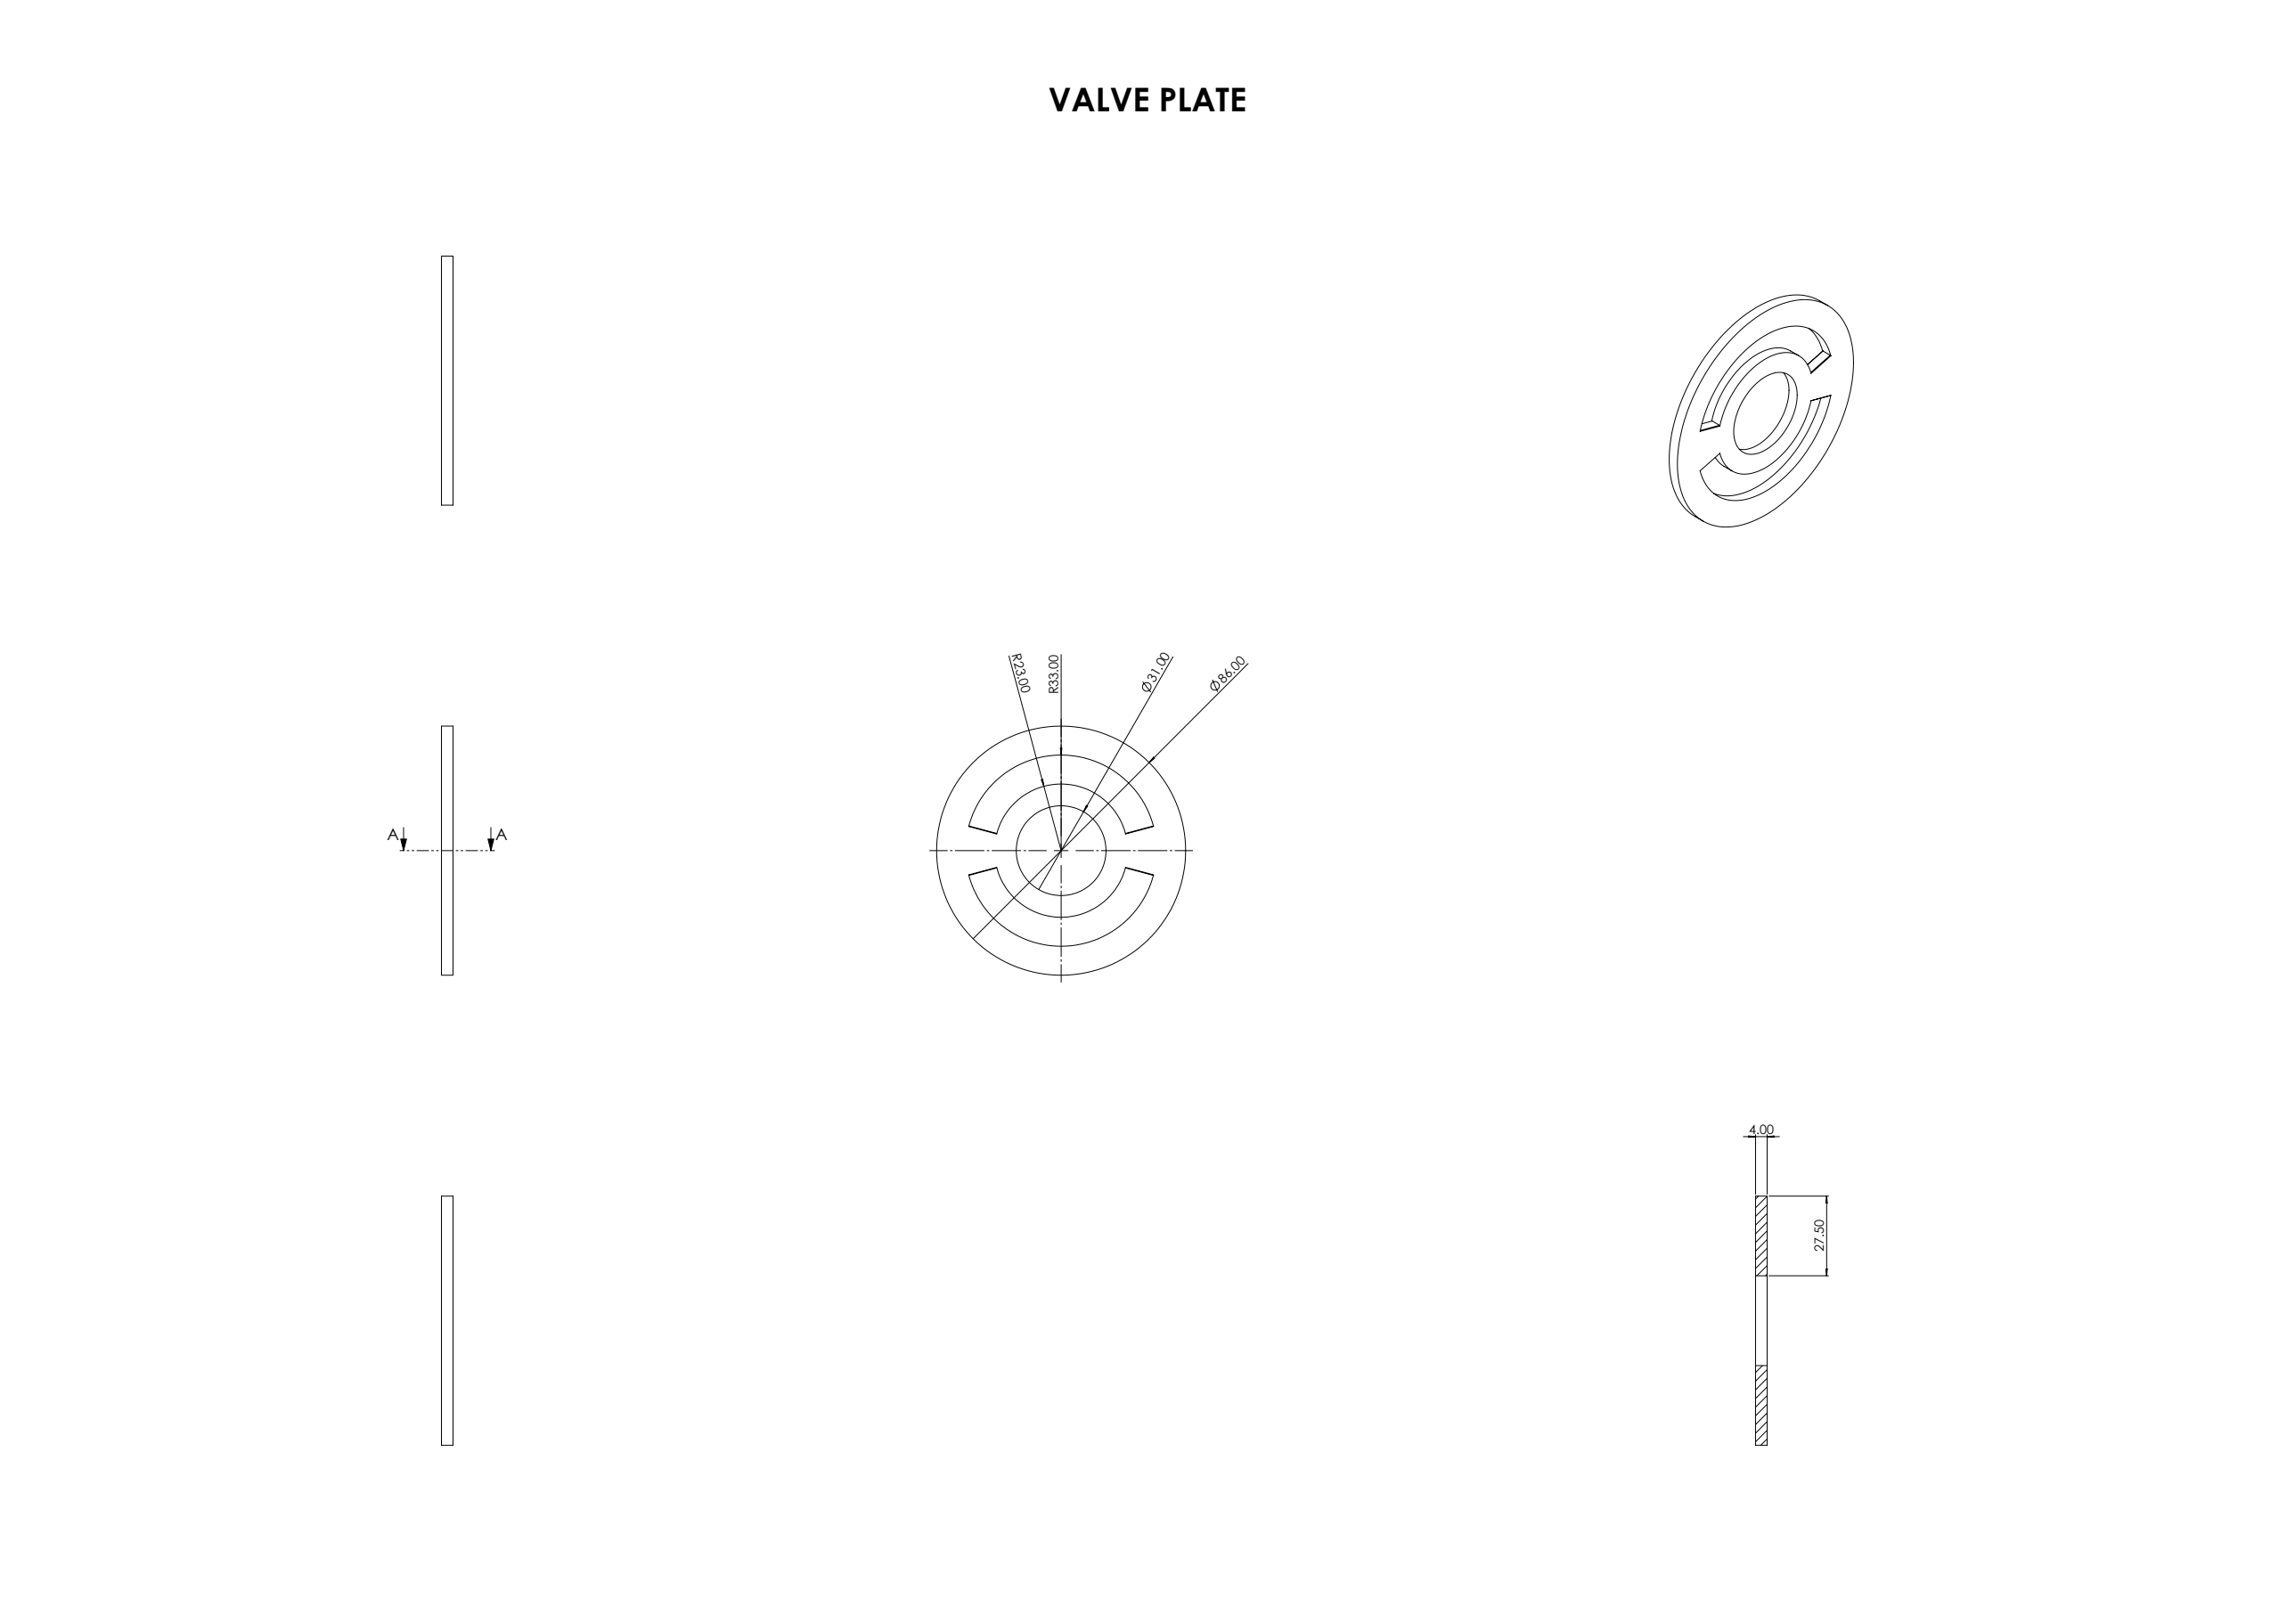
ISO-10303-21;
HEADER;
/* Generated by software containing ST-Developer
 * from STEP Tools, Inc. (www.steptools.com) 
 */

FILE_DESCRIPTION(
/* description */ (''),
/* implementation_level */ '2;1');

FILE_NAME(
/* name */ '08_Valve_Plate.step',
/* time_stamp */ '2026-10-26T07:49:00-07:00',
/* author */ (''),
/* organization */ (''),
/* preprocessor_version */ 'ST-DEVELOPER v20.2',
/* originating_system */ 'Autodesk Translation Framework v15.15.0.0',
/* authorisation */ '');

FILE_SCHEMA (('AUTOMOTIVE_DESIGN { 1 0 10303 214 3 1 1 }'));
ENDSEC;

DATA;
#10=MECHANICAL_DESIGN_GEOMETRIC_PRESENTATION_REPRESENTATION('',(#181),#38507);
#151=SHAPE_REPRESENTATION_RELATIONSHIP('SRR','None',#38579,#166);
#166=ADVANCED_BREP_SHAPE_REPRESENTATION('',(#196),#38496);
#181=STYLED_ITEM('',(#38706),#196);
#196=MANIFOLD_SOLID_BREP('Body1',#15075);
#316=ELLIPSE('',#15903,32.5269119345808,23.);
#317=ELLIPSE('',#15904,46.6690475583115,33.);
#318=ELLIPSE('',#15907,46.6690475583112,33.);
#319=ELLIPSE('',#15908,32.5269119345805,23.);
#320=ELLIPSE('',#15910,46.6690475583115,33.);
#321=ELLIPSE('',#15911,32.5269119345807,23.);
#322=ELLIPSE('',#15914,32.5269119345808,23.);
#323=ELLIPSE('',#15915,46.6690475583116,33.);
#324=ELLIPSE('',#15917,32.5269119345811,23.);
#325=ELLIPSE('',#15918,46.669047558312,33.);
#326=ELLIPSE('',#15921,46.669047558312,33.);
#327=ELLIPSE('',#15922,32.5269119345811,23.);
#328=ELLIPSE('',#15924,46.6690475583117,33.);
#329=ELLIPSE('',#15925,32.5269119345809,23.);
#330=ELLIPSE('',#15928,32.5269119345811,23.);
#331=ELLIPSE('',#15929,46.669047558312,33.);
#480=FACE_BOUND('',#2926,.T.);
#481=FACE_BOUND('',#2927,.T.);
#482=FACE_BOUND('',#2928,.T.);
#483=FACE_BOUND('',#2931,.T.);
#484=FACE_BOUND('',#2932,.T.);
#485=FACE_BOUND('',#2933,.T.);
#652=PLANE('',#15902);
#653=PLANE('',#15905);
#654=PLANE('',#15906);
#655=PLANE('',#15909);
#656=PLANE('',#15912);
#657=PLANE('',#15913);
#658=PLANE('',#15916);
#659=PLANE('',#15919);
#660=PLANE('',#15920);
#661=PLANE('',#15923);
#662=PLANE('',#15926);
#663=PLANE('',#15927);
#664=PLANE('',#15945);
#665=PLANE('',#15949);
#1483=CYLINDRICAL_SURFACE('',#15930,33.);
#1484=CYLINDRICAL_SURFACE('',#15933,23.);
#1485=CYLINDRICAL_SURFACE('',#15936,33.);
#1486=CYLINDRICAL_SURFACE('',#15939,23.);
#1487=CYLINDRICAL_SURFACE('',#15942,15.5);
#1488=CYLINDRICAL_SURFACE('',#15947,43.);
#1958=FACE_OUTER_BOUND('',#2908,.T.);
#1959=FACE_OUTER_BOUND('',#2909,.T.);
#1960=FACE_OUTER_BOUND('',#2910,.T.);
#1961=FACE_OUTER_BOUND('',#2911,.T.);
#1962=FACE_OUTER_BOUND('',#2912,.T.);
#1963=FACE_OUTER_BOUND('',#2913,.T.);
#1964=FACE_OUTER_BOUND('',#2914,.T.);
#1965=FACE_OUTER_BOUND('',#2915,.T.);
#1966=FACE_OUTER_BOUND('',#2916,.T.);
#1967=FACE_OUTER_BOUND('',#2917,.T.);
#1968=FACE_OUTER_BOUND('',#2918,.T.);
#1969=FACE_OUTER_BOUND('',#2919,.T.);
#1970=FACE_OUTER_BOUND('',#2920,.T.);
#1971=FACE_OUTER_BOUND('',#2921,.T.);
#1972=FACE_OUTER_BOUND('',#2922,.T.);
#1973=FACE_OUTER_BOUND('',#2923,.T.);
#1974=FACE_OUTER_BOUND('',#2924,.T.);
#1975=FACE_OUTER_BOUND('',#2925,.T.);
#1976=FACE_OUTER_BOUND('',#2929,.T.);
#1977=FACE_OUTER_BOUND('',#2930,.T.);
#2908=EDGE_LOOP('',(#11389,#11390,#11391,#11392));
#2909=EDGE_LOOP('',(#11393,#11394,#11395,#11396));
#2910=EDGE_LOOP('',(#11397,#11398,#11399,#11400));
#2911=EDGE_LOOP('',(#11401,#11402,#11403,#11404));
#2912=EDGE_LOOP('',(#11405,#11406,#11407,#11408));
#2913=EDGE_LOOP('',(#11409,#11410,#11411,#11412));
#2914=EDGE_LOOP('',(#11413,#11414,#11415,#11416));
#2915=EDGE_LOOP('',(#11417,#11418,#11419,#11420));
#2916=EDGE_LOOP('',(#11421,#11422,#11423,#11424));
#2917=EDGE_LOOP('',(#11425,#11426,#11427,#11428));
#2918=EDGE_LOOP('',(#11429,#11430,#11431,#11432));
#2919=EDGE_LOOP('',(#11433,#11434,#11435,#11436));
#2920=EDGE_LOOP('',(#11437,#11438,#11439,#11440,#11441,#11442,#11443,#11444));
#2921=EDGE_LOOP('',(#11445,#11446,#11447,#11448,#11449,#11450,#11451,#11452));
#2922=EDGE_LOOP('',(#11453,#11454,#11455,#11456,#11457,#11458,#11459,#11460));
#2923=EDGE_LOOP('',(#11461,#11462,#11463,#11464,#11465,#11466,#11467,#11468));
#2924=EDGE_LOOP('',(#11469,#11470,#11471,#11472));
#2925=EDGE_LOOP('',(#11473));
#2926=EDGE_LOOP('',(#11474,#11475,#11476,#11477));
#2927=EDGE_LOOP('',(#11478,#11479,#11480,#11481));
#2928=EDGE_LOOP('',(#11482));
#2929=EDGE_LOOP('',(#11483,#11484,#11485,#11486));
#2930=EDGE_LOOP('',(#11487));
#2931=EDGE_LOOP('',(#11488,#11489,#11490,#11491));
#2932=EDGE_LOOP('',(#11492,#11493,#11494,#11495));
#2933=EDGE_LOOP('',(#11496));
#3820=LINE('',#25636,#4889);
#3821=LINE('',#25639,#4890);
#3822=LINE('',#25642,#4891);
#3823=LINE('',#25644,#4892);
#3824=LINE('',#25645,#4893);
#3825=LINE('',#25651,#4894);
#3826=LINE('',#25657,#4895);
#3827=LINE('',#25660,#4896);
#3828=LINE('',#25663,#4897);
#3829=LINE('',#25665,#4898);
#3830=LINE('',#25666,#4899);
#3831=LINE('',#25672,#4900);
#3832=LINE('',#25678,#4901);
#3833=LINE('',#25681,#4902);
#3834=LINE('',#25684,#4903);
#3835=LINE('',#25686,#4904);
#3836=LINE('',#25687,#4905);
#3837=LINE('',#25693,#4906);
#3838=LINE('',#25699,#4907);
#3839=LINE('',#25702,#4908);
#3840=LINE('',#25705,#4909);
#3841=LINE('',#25707,#4910);
#3842=LINE('',#25708,#4911);
#3843=LINE('',#25714,#4912);
#3844=LINE('',#25731,#4913);
#3845=LINE('',#25739,#4914);
#4889=VECTOR('',#18367,10.);
#4890=VECTOR('',#18370,10.);
#4891=VECTOR('',#18373,10.);
#4892=VECTOR('',#18374,10.);
#4893=VECTOR('',#18375,10.);
#4894=VECTOR('',#18382,10.);
#4895=VECTOR('',#18387,10.);
#4896=VECTOR('',#18390,10.);
#4897=VECTOR('',#18393,10.);
#4898=VECTOR('',#18394,10.);
#4899=VECTOR('',#18395,10.);
#4900=VECTOR('',#18402,10.);
#4901=VECTOR('',#18407,10.);
#4902=VECTOR('',#18410,10.);
#4903=VECTOR('',#18413,10.);
#4904=VECTOR('',#18414,10.);
#4905=VECTOR('',#18415,10.);
#4906=VECTOR('',#18422,10.);
#4907=VECTOR('',#18427,10.);
#4908=VECTOR('',#18430,10.);
#4909=VECTOR('',#18433,10.);
#4910=VECTOR('',#18434,10.);
#4911=VECTOR('',#18435,10.);
#4912=VECTOR('',#18442,10.);
#4913=VECTOR('',#18471,15.5);
#4914=VECTOR('',#18482,43.);
#5995=CIRCLE('',#15931,33.);
#5996=CIRCLE('',#15932,33.);
#5997=CIRCLE('',#15934,23.);
#5998=CIRCLE('',#15935,23.);
#5999=CIRCLE('',#15937,33.);
#6000=CIRCLE('',#15938,33.);
#6001=CIRCLE('',#15940,23.);
#6002=CIRCLE('',#15941,23.);
#6003=CIRCLE('',#15943,15.5);
#6004=CIRCLE('',#15944,15.5);
#6005=CIRCLE('',#15946,43.);
#6006=CIRCLE('',#15948,43.);
#6756=VERTEX_POINT('',#25632);
#6757=VERTEX_POINT('',#25633);
#6758=VERTEX_POINT('',#25635);
#6759=VERTEX_POINT('',#25637);
#6760=VERTEX_POINT('',#25641);
#6761=VERTEX_POINT('',#25643);
#6762=VERTEX_POINT('',#25647);
#6763=VERTEX_POINT('',#25649);
#6764=VERTEX_POINT('',#25653);
#6765=VERTEX_POINT('',#25654);
#6766=VERTEX_POINT('',#25656);
#6767=VERTEX_POINT('',#25658);
#6768=VERTEX_POINT('',#25662);
#6769=VERTEX_POINT('',#25664);
#6770=VERTEX_POINT('',#25668);
#6771=VERTEX_POINT('',#25670);
#6772=VERTEX_POINT('',#25674);
#6773=VERTEX_POINT('',#25675);
#6774=VERTEX_POINT('',#25677);
#6775=VERTEX_POINT('',#25679);
#6776=VERTEX_POINT('',#25683);
#6777=VERTEX_POINT('',#25685);
#6778=VERTEX_POINT('',#25689);
#6779=VERTEX_POINT('',#25691);
#6780=VERTEX_POINT('',#25695);
#6781=VERTEX_POINT('',#25696);
#6782=VERTEX_POINT('',#25698);
#6783=VERTEX_POINT('',#25700);
#6784=VERTEX_POINT('',#25704);
#6785=VERTEX_POINT('',#25706);
#6786=VERTEX_POINT('',#25710);
#6787=VERTEX_POINT('',#25712);
#6788=VERTEX_POINT('',#25728);
#6789=VERTEX_POINT('',#25730);
#6790=VERTEX_POINT('',#25734);
#6791=VERTEX_POINT('',#25737);
#8443=EDGE_CURVE('',#6756,#6757,#316,.F.);
#8444=EDGE_CURVE('',#6757,#6758,#3820,.T.);
#8445=EDGE_CURVE('',#6758,#6759,#317,.F.);
#8446=EDGE_CURVE('',#6759,#6756,#3821,.T.);
#8447=EDGE_CURVE('',#6760,#6757,#3822,.T.);
#8448=EDGE_CURVE('',#6761,#6760,#3823,.T.);
#8449=EDGE_CURVE('',#6761,#6758,#3824,.T.);
#8450=EDGE_CURVE('',#6762,#6761,#318,.F.);
#8451=EDGE_CURVE('',#6760,#6763,#319,.F.);
#8452=EDGE_CURVE('',#6763,#6762,#3825,.T.);
#8453=EDGE_CURVE('',#6764,#6765,#320,.F.);
#8454=EDGE_CURVE('',#6765,#6766,#3826,.T.);
#8455=EDGE_CURVE('',#6766,#6767,#321,.F.);
#8456=EDGE_CURVE('',#6767,#6764,#3827,.T.);
#8457=EDGE_CURVE('',#6768,#6765,#3828,.T.);
#8458=EDGE_CURVE('',#6769,#6768,#3829,.T.);
#8459=EDGE_CURVE('',#6769,#6766,#3830,.T.);
#8460=EDGE_CURVE('',#6770,#6769,#322,.F.);
#8461=EDGE_CURVE('',#6768,#6771,#323,.F.);
#8462=EDGE_CURVE('',#6771,#6770,#3831,.T.);
#8463=EDGE_CURVE('',#6772,#6773,#324,.F.);
#8464=EDGE_CURVE('',#6773,#6774,#3832,.T.);
#8465=EDGE_CURVE('',#6774,#6775,#325,.F.);
#8466=EDGE_CURVE('',#6775,#6772,#3833,.T.);
#8467=EDGE_CURVE('',#6776,#6773,#3834,.T.);
#8468=EDGE_CURVE('',#6777,#6776,#3835,.T.);
#8469=EDGE_CURVE('',#6777,#6774,#3836,.T.);
#8470=EDGE_CURVE('',#6778,#6777,#326,.F.);
#8471=EDGE_CURVE('',#6776,#6779,#327,.F.);
#8472=EDGE_CURVE('',#6779,#6778,#3837,.T.);
#8473=EDGE_CURVE('',#6780,#6781,#328,.F.);
#8474=EDGE_CURVE('',#6781,#6782,#3838,.T.);
#8475=EDGE_CURVE('',#6782,#6783,#329,.F.);
#8476=EDGE_CURVE('',#6783,#6780,#3839,.T.);
#8477=EDGE_CURVE('',#6784,#6781,#3840,.T.);
#8478=EDGE_CURVE('',#6785,#6784,#3841,.T.);
#8479=EDGE_CURVE('',#6785,#6782,#3842,.T.);
#8480=EDGE_CURVE('',#6786,#6785,#330,.F.);
#8481=EDGE_CURVE('',#6784,#6787,#331,.F.);
#8482=EDGE_CURVE('',#6787,#6786,#3843,.T.);
#8483=EDGE_CURVE('',#6787,#6778,#5995,.T.);
#8484=EDGE_CURVE('',#6775,#6780,#5996,.T.);
#8485=EDGE_CURVE('',#6779,#6786,#5997,.T.);
#8486=EDGE_CURVE('',#6783,#6772,#5998,.T.);
#8487=EDGE_CURVE('',#6771,#6762,#5999,.T.);
#8488=EDGE_CURVE('',#6759,#6764,#6000,.T.);
#8489=EDGE_CURVE('',#6763,#6770,#6001,.T.);
#8490=EDGE_CURVE('',#6767,#6756,#6002,.T.);
#8491=EDGE_CURVE('',#6788,#6788,#6003,.T.);
#8492=EDGE_CURVE('',#6788,#6789,#3844,.T.);
#8493=EDGE_CURVE('',#6789,#6789,#6004,.T.);
#8494=EDGE_CURVE('',#6790,#6790,#6005,.T.);
#8495=EDGE_CURVE('',#6791,#6791,#6006,.T.);
#8496=EDGE_CURVE('',#6791,#6790,#3845,.T.);
#11389=ORIENTED_EDGE('',*,*,#8443,.T.);
#11390=ORIENTED_EDGE('',*,*,#8444,.T.);
#11391=ORIENTED_EDGE('',*,*,#8445,.T.);
#11392=ORIENTED_EDGE('',*,*,#8446,.T.);
#11393=ORIENTED_EDGE('',*,*,#8444,.F.);
#11394=ORIENTED_EDGE('',*,*,#8447,.F.);
#11395=ORIENTED_EDGE('',*,*,#8448,.F.);
#11396=ORIENTED_EDGE('',*,*,#8449,.T.);
#11397=ORIENTED_EDGE('',*,*,#8450,.T.);
#11398=ORIENTED_EDGE('',*,*,#8448,.T.);
#11399=ORIENTED_EDGE('',*,*,#8451,.T.);
#11400=ORIENTED_EDGE('',*,*,#8452,.T.);
#11401=ORIENTED_EDGE('',*,*,#8453,.T.);
#11402=ORIENTED_EDGE('',*,*,#8454,.T.);
#11403=ORIENTED_EDGE('',*,*,#8455,.T.);
#11404=ORIENTED_EDGE('',*,*,#8456,.T.);
#11405=ORIENTED_EDGE('',*,*,#8454,.F.);
#11406=ORIENTED_EDGE('',*,*,#8457,.F.);
#11407=ORIENTED_EDGE('',*,*,#8458,.F.);
#11408=ORIENTED_EDGE('',*,*,#8459,.T.);
#11409=ORIENTED_EDGE('',*,*,#8460,.T.);
#11410=ORIENTED_EDGE('',*,*,#8458,.T.);
#11411=ORIENTED_EDGE('',*,*,#8461,.T.);
#11412=ORIENTED_EDGE('',*,*,#8462,.T.);
#11413=ORIENTED_EDGE('',*,*,#8463,.T.);
#11414=ORIENTED_EDGE('',*,*,#8464,.T.);
#11415=ORIENTED_EDGE('',*,*,#8465,.T.);
#11416=ORIENTED_EDGE('',*,*,#8466,.T.);
#11417=ORIENTED_EDGE('',*,*,#8464,.F.);
#11418=ORIENTED_EDGE('',*,*,#8467,.F.);
#11419=ORIENTED_EDGE('',*,*,#8468,.F.);
#11420=ORIENTED_EDGE('',*,*,#8469,.T.);
#11421=ORIENTED_EDGE('',*,*,#8470,.T.);
#11422=ORIENTED_EDGE('',*,*,#8468,.T.);
#11423=ORIENTED_EDGE('',*,*,#8471,.T.);
#11424=ORIENTED_EDGE('',*,*,#8472,.T.);
#11425=ORIENTED_EDGE('',*,*,#8473,.T.);
#11426=ORIENTED_EDGE('',*,*,#8474,.T.);
#11427=ORIENTED_EDGE('',*,*,#8475,.T.);
#11428=ORIENTED_EDGE('',*,*,#8476,.T.);
#11429=ORIENTED_EDGE('',*,*,#8474,.F.);
#11430=ORIENTED_EDGE('',*,*,#8477,.F.);
#11431=ORIENTED_EDGE('',*,*,#8478,.F.);
#11432=ORIENTED_EDGE('',*,*,#8479,.T.);
#11433=ORIENTED_EDGE('',*,*,#8480,.T.);
#11434=ORIENTED_EDGE('',*,*,#8478,.T.);
#11435=ORIENTED_EDGE('',*,*,#8481,.T.);
#11436=ORIENTED_EDGE('',*,*,#8482,.T.);
#11437=ORIENTED_EDGE('',*,*,#8483,.F.);
#11438=ORIENTED_EDGE('',*,*,#8481,.F.);
#11439=ORIENTED_EDGE('',*,*,#8477,.T.);
#11440=ORIENTED_EDGE('',*,*,#8473,.F.);
#11441=ORIENTED_EDGE('',*,*,#8484,.F.);
#11442=ORIENTED_EDGE('',*,*,#8465,.F.);
#11443=ORIENTED_EDGE('',*,*,#8469,.F.);
#11444=ORIENTED_EDGE('',*,*,#8470,.F.);
#11445=ORIENTED_EDGE('',*,*,#8485,.F.);
#11446=ORIENTED_EDGE('',*,*,#8471,.F.);
#11447=ORIENTED_EDGE('',*,*,#8467,.T.);
#11448=ORIENTED_EDGE('',*,*,#8463,.F.);
#11449=ORIENTED_EDGE('',*,*,#8486,.F.);
#11450=ORIENTED_EDGE('',*,*,#8475,.F.);
#11451=ORIENTED_EDGE('',*,*,#8479,.F.);
#11452=ORIENTED_EDGE('',*,*,#8480,.F.);
#11453=ORIENTED_EDGE('',*,*,#8487,.F.);
#11454=ORIENTED_EDGE('',*,*,#8461,.F.);
#11455=ORIENTED_EDGE('',*,*,#8457,.T.);
#11456=ORIENTED_EDGE('',*,*,#8453,.F.);
#11457=ORIENTED_EDGE('',*,*,#8488,.F.);
#11458=ORIENTED_EDGE('',*,*,#8445,.F.);
#11459=ORIENTED_EDGE('',*,*,#8449,.F.);
#11460=ORIENTED_EDGE('',*,*,#8450,.F.);
#11461=ORIENTED_EDGE('',*,*,#8489,.F.);
#11462=ORIENTED_EDGE('',*,*,#8451,.F.);
#11463=ORIENTED_EDGE('',*,*,#8447,.T.);
#11464=ORIENTED_EDGE('',*,*,#8443,.F.);
#11465=ORIENTED_EDGE('',*,*,#8490,.F.);
#11466=ORIENTED_EDGE('',*,*,#8455,.F.);
#11467=ORIENTED_EDGE('',*,*,#8459,.F.);
#11468=ORIENTED_EDGE('',*,*,#8460,.F.);
#11469=ORIENTED_EDGE('',*,*,#8491,.T.);
#11470=ORIENTED_EDGE('',*,*,#8492,.T.);
#11471=ORIENTED_EDGE('',*,*,#8493,.F.);
#11472=ORIENTED_EDGE('',*,*,#8492,.F.);
#11473=ORIENTED_EDGE('',*,*,#8494,.F.);
#11474=ORIENTED_EDGE('',*,*,#8489,.T.);
#11475=ORIENTED_EDGE('',*,*,#8462,.F.);
#11476=ORIENTED_EDGE('',*,*,#8487,.T.);
#11477=ORIENTED_EDGE('',*,*,#8452,.F.);
#11478=ORIENTED_EDGE('',*,*,#8485,.T.);
#11479=ORIENTED_EDGE('',*,*,#8482,.F.);
#11480=ORIENTED_EDGE('',*,*,#8483,.T.);
#11481=ORIENTED_EDGE('',*,*,#8472,.F.);
#11482=ORIENTED_EDGE('',*,*,#8493,.T.);
#11483=ORIENTED_EDGE('',*,*,#8495,.F.);
#11484=ORIENTED_EDGE('',*,*,#8496,.T.);
#11485=ORIENTED_EDGE('',*,*,#8494,.T.);
#11486=ORIENTED_EDGE('',*,*,#8496,.F.);
#11487=ORIENTED_EDGE('',*,*,#8495,.T.);
#11488=ORIENTED_EDGE('',*,*,#8488,.T.);
#11489=ORIENTED_EDGE('',*,*,#8456,.F.);
#11490=ORIENTED_EDGE('',*,*,#8490,.T.);
#11491=ORIENTED_EDGE('',*,*,#8446,.F.);
#11492=ORIENTED_EDGE('',*,*,#8484,.T.);
#11493=ORIENTED_EDGE('',*,*,#8476,.F.);
#11494=ORIENTED_EDGE('',*,*,#8486,.T.);
#11495=ORIENTED_EDGE('',*,*,#8466,.F.);
#11496=ORIENTED_EDGE('',*,*,#8491,.F.);
#14525=ADVANCED_FACE('',(#1958),#652,.T.);
#14526=ADVANCED_FACE('',(#1959),#653,.F.);
#14527=ADVANCED_FACE('',(#1960),#654,.T.);
#14528=ADVANCED_FACE('',(#1961),#655,.T.);
#14529=ADVANCED_FACE('',(#1962),#656,.F.);
#14530=ADVANCED_FACE('',(#1963),#657,.T.);
#14531=ADVANCED_FACE('',(#1964),#658,.T.);
#14532=ADVANCED_FACE('',(#1965),#659,.F.);
#14533=ADVANCED_FACE('',(#1966),#660,.T.);
#14534=ADVANCED_FACE('',(#1967),#661,.T.);
#14535=ADVANCED_FACE('',(#1968),#662,.F.);
#14536=ADVANCED_FACE('',(#1969),#663,.T.);
#14537=ADVANCED_FACE('',(#1970),#1483,.F.);
#14538=ADVANCED_FACE('',(#1971),#1484,.T.);
#14539=ADVANCED_FACE('',(#1972),#1485,.F.);
#14540=ADVANCED_FACE('',(#1973),#1486,.T.);
#14541=ADVANCED_FACE('',(#1974),#1487,.F.);
#14542=ADVANCED_FACE('',(#1975,#480,#481,#482),#664,.T.);
#14543=ADVANCED_FACE('',(#1976),#1488,.T.);
#14544=ADVANCED_FACE('',(#1977,#483,#484,#485),#665,.T.);
#15075=CLOSED_SHELL('',(#14525,#14526,#14527,#14528,#14529,#14530,#14531,
#14532,#14533,#14534,#14535,#14536,#14537,#14538,#14539,#14540,#14541,#14542,
#14543,#14544));
#15901=AXIS2_PLACEMENT_3D('',#25630,#18361,#18362);
#15902=AXIS2_PLACEMENT_3D('',#25631,#18363,#18364);
#15903=AXIS2_PLACEMENT_3D('',#25634,#18365,#18366);
#15904=AXIS2_PLACEMENT_3D('',#25638,#18368,#18369);
#15905=AXIS2_PLACEMENT_3D('',#25640,#18371,#18372);
#15906=AXIS2_PLACEMENT_3D('',#25646,#18376,#18377);
#15907=AXIS2_PLACEMENT_3D('',#25648,#18378,#18379);
#15908=AXIS2_PLACEMENT_3D('',#25650,#18380,#18381);
#15909=AXIS2_PLACEMENT_3D('',#25652,#18383,#18384);
#15910=AXIS2_PLACEMENT_3D('',#25655,#18385,#18386);
#15911=AXIS2_PLACEMENT_3D('',#25659,#18388,#18389);
#15912=AXIS2_PLACEMENT_3D('',#25661,#18391,#18392);
#15913=AXIS2_PLACEMENT_3D('',#25667,#18396,#18397);
#15914=AXIS2_PLACEMENT_3D('',#25669,#18398,#18399);
#15915=AXIS2_PLACEMENT_3D('',#25671,#18400,#18401);
#15916=AXIS2_PLACEMENT_3D('',#25673,#18403,#18404);
#15917=AXIS2_PLACEMENT_3D('',#25676,#18405,#18406);
#15918=AXIS2_PLACEMENT_3D('',#25680,#18408,#18409);
#15919=AXIS2_PLACEMENT_3D('',#25682,#18411,#18412);
#15920=AXIS2_PLACEMENT_3D('',#25688,#18416,#18417);
#15921=AXIS2_PLACEMENT_3D('',#25690,#18418,#18419);
#15922=AXIS2_PLACEMENT_3D('',#25692,#18420,#18421);
#15923=AXIS2_PLACEMENT_3D('',#25694,#18423,#18424);
#15924=AXIS2_PLACEMENT_3D('',#25697,#18425,#18426);
#15925=AXIS2_PLACEMENT_3D('',#25701,#18428,#18429);
#15926=AXIS2_PLACEMENT_3D('',#25703,#18431,#18432);
#15927=AXIS2_PLACEMENT_3D('',#25709,#18436,#18437);
#15928=AXIS2_PLACEMENT_3D('',#25711,#18438,#18439);
#15929=AXIS2_PLACEMENT_3D('',#25713,#18440,#18441);
#15930=AXIS2_PLACEMENT_3D('',#25715,#18443,#18444);
#15931=AXIS2_PLACEMENT_3D('',#25716,#18445,#18446);
#15932=AXIS2_PLACEMENT_3D('',#25717,#18447,#18448);
#15933=AXIS2_PLACEMENT_3D('',#25718,#18449,#18450);
#15934=AXIS2_PLACEMENT_3D('',#25719,#18451,#18452);
#15935=AXIS2_PLACEMENT_3D('',#25720,#18453,#18454);
#15936=AXIS2_PLACEMENT_3D('',#25721,#18455,#18456);
#15937=AXIS2_PLACEMENT_3D('',#25722,#18457,#18458);
#15938=AXIS2_PLACEMENT_3D('',#25723,#18459,#18460);
#15939=AXIS2_PLACEMENT_3D('',#25724,#18461,#18462);
#15940=AXIS2_PLACEMENT_3D('',#25725,#18463,#18464);
#15941=AXIS2_PLACEMENT_3D('',#25726,#18465,#18466);
#15942=AXIS2_PLACEMENT_3D('',#25727,#18467,#18468);
#15943=AXIS2_PLACEMENT_3D('',#25729,#18469,#18470);
#15944=AXIS2_PLACEMENT_3D('',#25732,#18472,#18473);
#15945=AXIS2_PLACEMENT_3D('',#25733,#18474,#18475);
#15946=AXIS2_PLACEMENT_3D('',#25735,#18476,#18477);
#15947=AXIS2_PLACEMENT_3D('',#25736,#18478,#18479);
#15948=AXIS2_PLACEMENT_3D('',#25738,#18480,#18481);
#15949=AXIS2_PLACEMENT_3D('',#25740,#18483,#18484);
#18361=DIRECTION('axis',(0.,0.,1.));
#18362=DIRECTION('refdir',(1.,0.,0.));
#18363=DIRECTION('center_axis',(0.707106781186557,0.68301270189221,-0.183012701892217));
#18364=DIRECTION('ref_axis',(-0.250562807085725,0.,-0.968100345886377));
#18365=DIRECTION('center_axis',(0.707106781186557,0.68301270189221,-0.183012701892217));
#18366=DIRECTION('ref_axis',(-0.707106781186538,0.683012701892228,-0.183012701892222));
#18367=DIRECTION('',(0.,0.258819045102521,0.965925826289068));
#18368=DIRECTION('center_axis',(-0.707106781186557,-0.68301270189221,0.183012701892217));
#18369=DIRECTION('ref_axis',(-0.707106781186538,0.683012701892229,-0.183012701892222));
#18370=DIRECTION('',(0.,-0.258819045102521,-0.965925826289068));
#18371=DIRECTION('center_axis',(0.,-0.965925826289068,0.258819045102521));
#18372=DIRECTION('ref_axis',(0.,-0.258819045102521,-0.965925826289068));
#18373=DIRECTION('',(1.,0.,0.));
#18374=DIRECTION('',(0.,-0.258819045102521,-0.965925826289068));
#18375=DIRECTION('',(1.,0.,0.));
#18376=DIRECTION('center_axis',(-0.707106781186562,0.683012701892206,-0.183012701892215));
#18377=DIRECTION('ref_axis',(-0.250562807085722,0.,0.968100345886377));
#18378=DIRECTION('center_axis',(0.707106781186562,-0.683012701892206,0.183012701892215));
#18379=DIRECTION('ref_axis',(0.707106781186533,0.683012701892233,-0.183012701892223));
#18380=DIRECTION('center_axis',(-0.707106781186562,0.683012701892206,-0.183012701892215));
#18381=DIRECTION('ref_axis',(0.707106781186533,0.683012701892233,-0.183012701892223));
#18382=DIRECTION('',(0.,0.258819045102521,0.965925826289068));
#18383=DIRECTION('center_axis',(0.707106781186557,0.68301270189221,0.183012701892217));
#18384=DIRECTION('ref_axis',(0.250562807085726,0.,-0.968100345886376));
#18385=DIRECTION('center_axis',(-0.707106781186557,-0.68301270189221,-0.183012701892217));
#18386=DIRECTION('ref_axis',(-0.707106781186538,0.683012701892228,0.183012701892222));
#18387=DIRECTION('',(0.,-0.258819045102521,0.965925826289068));
#18388=DIRECTION('center_axis',(0.707106781186557,0.68301270189221,0.183012701892217));
#18389=DIRECTION('ref_axis',(-0.707106781186538,0.683012701892229,0.183012701892222));
#18390=DIRECTION('',(0.,0.258819045102521,-0.965925826289068));
#18391=DIRECTION('center_axis',(0.,-0.965925826289068,-0.258819045102521));
#18392=DIRECTION('ref_axis',(0.,0.258819045102521,-0.965925826289068));
#18393=DIRECTION('',(1.,0.,0.));
#18394=DIRECTION('',(0.,0.258819045102521,-0.965925826289068));
#18395=DIRECTION('',(1.,0.,0.));
#18396=DIRECTION('center_axis',(-0.707106781186556,0.683012701892211,0.183012701892217));
#18397=DIRECTION('ref_axis',(0.250562807085726,0.,0.968100345886376));
#18398=DIRECTION('center_axis',(-0.707106781186556,0.683012701892211,0.183012701892217));
#18399=DIRECTION('ref_axis',(0.707106781186539,0.683012701892228,0.183012701892222));
#18400=DIRECTION('center_axis',(0.707106781186556,-0.683012701892211,-0.183012701892217));
#18401=DIRECTION('ref_axis',(0.707106781186539,0.683012701892228,0.183012701892222));
#18402=DIRECTION('',(0.,-0.258819045102521,0.965925826289068));
#18403=DIRECTION('center_axis',(0.70710678118655,-0.683012701892217,0.183012701892219));
#18404=DIRECTION('ref_axis',(0.25056280708573,0.,-0.968100345886375));
#18405=DIRECTION('center_axis',(0.70710678118655,-0.683012701892217,0.183012701892219));
#18406=DIRECTION('ref_axis',(-0.707106781186545,-0.683012701892222,0.18301270189222));
#18407=DIRECTION('',(0.,-0.258819045102521,-0.965925826289068));
#18408=DIRECTION('center_axis',(-0.70710678118655,0.683012701892217,-0.183012701892219));
#18409=DIRECTION('ref_axis',(-0.707106781186545,-0.683012701892222,0.18301270189222));
#18410=DIRECTION('',(0.,0.258819045102521,0.965925826289068));
#18411=DIRECTION('center_axis',(0.,0.965925826289068,-0.258819045102521));
#18412=DIRECTION('ref_axis',(0.,0.258819045102521,0.965925826289068));
#18413=DIRECTION('',(1.,0.,0.));
#18414=DIRECTION('',(0.,0.258819045102521,0.965925826289068));
#18415=DIRECTION('',(1.,0.,0.));
#18416=DIRECTION('center_axis',(-0.70710678118655,-0.683012701892217,0.183012701892219));
#18417=DIRECTION('ref_axis',(0.25056280708573,0.,0.968100345886375));
#18418=DIRECTION('center_axis',(0.70710678118655,0.683012701892217,-0.183012701892219));
#18419=DIRECTION('ref_axis',(0.707106781186545,-0.683012701892222,0.18301270189222));
#18420=DIRECTION('center_axis',(-0.70710678118655,-0.683012701892217,0.183012701892219));
#18421=DIRECTION('ref_axis',(0.707106781186545,-0.683012701892222,0.18301270189222));
#18422=DIRECTION('',(0.,-0.258819045102521,-0.965925826289068));
#18423=DIRECTION('center_axis',(0.707106781186554,-0.683012701892213,-0.183012701892218));
#18424=DIRECTION('ref_axis',(-0.250562807085727,0.,-0.968100345886376));
#18425=DIRECTION('center_axis',(-0.707106781186554,0.683012701892213,0.183012701892218));
#18426=DIRECTION('ref_axis',(-0.707106781186541,-0.683012701892225,-0.183012701892221));
#18427=DIRECTION('',(0.,0.258819045102521,-0.965925826289068));
#18428=DIRECTION('center_axis',(0.707106781186554,-0.683012701892213,-0.183012701892218));
#18429=DIRECTION('ref_axis',(-0.707106781186541,-0.683012701892225,-0.183012701892221));
#18430=DIRECTION('',(0.,-0.258819045102521,0.965925826289068));
#18431=DIRECTION('center_axis',(0.,0.965925826289068,0.258819045102521));
#18432=DIRECTION('ref_axis',(0.,-0.258819045102521,0.965925826289068));
#18433=DIRECTION('',(1.,0.,0.));
#18434=DIRECTION('',(0.,-0.258819045102521,0.965925826289068));
#18435=DIRECTION('',(1.,0.,0.));
#18436=DIRECTION('center_axis',(-0.707106781186549,-0.683012701892218,-0.183012701892219));
#18437=DIRECTION('ref_axis',(-0.25056280708573,0.,0.968100345886375));
#18438=DIRECTION('center_axis',(-0.707106781186549,-0.683012701892218,-0.183012701892219));
#18439=DIRECTION('ref_axis',(0.707106781186546,-0.683012701892221,-0.18301270189222));
#18440=DIRECTION('center_axis',(0.707106781186549,0.683012701892218,0.183012701892219));
#18441=DIRECTION('ref_axis',(0.707106781186546,-0.683012701892221,-0.18301270189222));
#18442=DIRECTION('',(0.,0.258819045102521,-0.965925826289068));
#18443=DIRECTION('center_axis',(1.,0.,0.));
#18444=DIRECTION('ref_axis',(0.,-0.258819045102521,0.965925826289068));
#18445=DIRECTION('center_axis',(1.,0.,0.));
#18446=DIRECTION('ref_axis',(0.,-0.258819045102521,0.965925826289068));
#18447=DIRECTION('center_axis',(-1.,0.,0.));
#18448=DIRECTION('ref_axis',(0.,-0.258819045102521,0.965925826289068));
#18449=DIRECTION('center_axis',(1.,0.,0.));
#18450=DIRECTION('ref_axis',(0.,-0.258819045102521,0.965925826289068));
#18451=DIRECTION('center_axis',(-1.,0.,0.));
#18452=DIRECTION('ref_axis',(0.,-0.258819045102521,0.965925826289068));
#18453=DIRECTION('center_axis',(1.,0.,0.));
#18454=DIRECTION('ref_axis',(0.,-0.258819045102521,0.965925826289068));
#18455=DIRECTION('center_axis',(1.,0.,0.));
#18456=DIRECTION('ref_axis',(0.,0.258819045102521,-0.965925826289068));
#18457=DIRECTION('center_axis',(1.,0.,0.));
#18458=DIRECTION('ref_axis',(0.,0.258819045102521,-0.965925826289068));
#18459=DIRECTION('center_axis',(-1.,0.,0.));
#18460=DIRECTION('ref_axis',(0.,0.258819045102521,-0.965925826289068));
#18461=DIRECTION('center_axis',(1.,0.,0.));
#18462=DIRECTION('ref_axis',(0.,0.258819045102521,-0.965925826289068));
#18463=DIRECTION('center_axis',(-1.,0.,0.));
#18464=DIRECTION('ref_axis',(0.,0.258819045102521,-0.965925826289068));
#18465=DIRECTION('center_axis',(1.,0.,0.));
#18466=DIRECTION('ref_axis',(0.,0.258819045102521,-0.965925826289068));
#18467=DIRECTION('center_axis',(1.,0.,0.));
#18468=DIRECTION('ref_axis',(0.,1.,0.));
#18469=DIRECTION('center_axis',(1.,0.,0.));
#18470=DIRECTION('ref_axis',(0.,0.,-1.));
#18471=DIRECTION('',(-1.,0.,0.));
#18472=DIRECTION('center_axis',(1.,0.,0.));
#18473=DIRECTION('ref_axis',(0.,0.,-1.));
#18474=DIRECTION('center_axis',(-1.,0.,0.));
#18475=DIRECTION('ref_axis',(0.,0.,1.));
#18476=DIRECTION('center_axis',(1.,0.,0.));
#18477=DIRECTION('ref_axis',(0.,0.,-1.));
#18478=DIRECTION('center_axis',(1.,0.,0.));
#18479=DIRECTION('ref_axis',(0.,1.,0.));
#18480=DIRECTION('center_axis',(1.,0.,0.));
#18481=DIRECTION('ref_axis',(0.,0.,-1.));
#18482=DIRECTION('',(-1.,0.,0.));
#18483=DIRECTION('center_axis',(1.,0.,0.));
#18484=DIRECTION('ref_axis',(0.,0.,-1.));
#25630=CARTESIAN_POINT('',(0.,0.,0.));
#25631=CARTESIAN_POINT('Origin',(129.7,4.69307322189799,17.9011580382799));
#25632=CARTESIAN_POINT('',(129.8,5.75942780780634,22.2672178622896));
#25633=CARTESIAN_POINT('',(129.6,5.95283803735798,22.2162940046486));
#25634=CARTESIAN_POINT('Origin',(129.6,-2.22044604925031E-15,0.));
#25635=CARTESIAN_POINT('',(129.6,8.54102848838318,31.8755522675393));
#25636=CARTESIAN_POINT('',(129.6,4.78966580452689,17.8752761337696));
#25637=CARTESIAN_POINT('',(129.8,8.3476864616576,31.9267306615923));
#25638=CARTESIAN_POINT('Origin',(129.6,0.,4.44089209850063E-15));
#25639=CARTESIAN_POINT('',(129.8,4.59648063926908,17.9270399427901));
#25640=CARTESIAN_POINT('Origin',(125.8,8.54102848838318,31.8755522675393));
#25641=CARTESIAN_POINT('',(126.,5.95283803735798,22.2162940046486));
#25642=CARTESIAN_POINT('',(125.8,5.95283803735798,22.2162940046486));
#25643=CARTESIAN_POINT('',(126.,8.54102848838318,31.8755522675393));
#25644=CARTESIAN_POINT('',(126.,5.71074115350888,21.3127761337696));
#25645=CARTESIAN_POINT('',(125.8,8.54102848838318,31.8755522675393));
#25646=CARTESIAN_POINT('Origin',(125.9,5.61414857087997,21.3386580382799));
#25647=CARTESIAN_POINT('',(125.8,8.3476864616576,31.9267306615923));
#25648=CARTESIAN_POINT('Origin',(126.,0.,4.44089209850063E-15));
#25649=CARTESIAN_POINT('',(125.8,5.75942780780634,22.2672178622896));
#25650=CARTESIAN_POINT('Origin',(126.,-2.22044604925031E-15,0.));
#25651=CARTESIAN_POINT('',(125.8,5.51755598825106,21.3645399427901));
#25652=CARTESIAN_POINT('Origin',(129.7,3.39897799638539,-13.0715289068345));
#25653=CARTESIAN_POINT('',(129.8,8.34768646165761,-31.9267306615923));
#25654=CARTESIAN_POINT('',(129.6,8.54102848838319,-31.8755522675393));
#25655=CARTESIAN_POINT('Origin',(129.6,0.,4.44089209850063E-15));
#25656=CARTESIAN_POINT('',(129.6,5.95283803735798,-22.2162940046486));
#25657=CARTESIAN_POINT('',(129.6,3.49557057901429,-13.0456470023243));
#25658=CARTESIAN_POINT('',(129.8,5.75942780780635,-22.2672178622896));
#25659=CARTESIAN_POINT('Origin',(129.6,-2.22044604925031E-15,0.));
#25660=CARTESIAN_POINT('',(129.8,3.30238541375648,-13.0974108113448));
#25661=CARTESIAN_POINT('Origin',(125.8,5.95283803735798,-22.2162940046486));
#25662=CARTESIAN_POINT('',(126.,8.54102848838319,-31.8755522675393));
#25663=CARTESIAN_POINT('',(125.8,8.54102848838319,-31.8755522675393));
#25664=CARTESIAN_POINT('',(126.,5.95283803735798,-22.2162940046486));
#25665=CARTESIAN_POINT('',(126.,4.41664592799628,-16.4831470023243));
#25666=CARTESIAN_POINT('',(125.8,5.95283803735798,-22.2162940046486));
#25667=CARTESIAN_POINT('Origin',(125.9,4.32005334536737,-16.5090289068345));
#25668=CARTESIAN_POINT('',(125.8,5.75942780780635,-22.2672178622896));
#25669=CARTESIAN_POINT('Origin',(126.,-2.22044604925031E-15,0.));
#25670=CARTESIAN_POINT('',(125.8,8.34768646165761,-31.9267306615923));
#25671=CARTESIAN_POINT('Origin',(126.,0.,4.44089209850063E-15));
#25672=CARTESIAN_POINT('',(125.8,4.22346076273846,-16.5349108113448));
#25673=CARTESIAN_POINT('Origin',(129.7,-3.65477010122739,-14.0261580382799));
#25674=CARTESIAN_POINT('',(129.8,-5.75942780780635,-22.2672178622896));
#25675=CARTESIAN_POINT('',(129.6,-5.95283803735798,-22.2162940046486));
#25676=CARTESIAN_POINT('Origin',(129.6,0.,0.));
#25677=CARTESIAN_POINT('',(129.6,-8.54102848838319,-31.8755522675393));
#25678=CARTESIAN_POINT('',(129.6,-3.75136268385629,-14.0002761337696));
#25679=CARTESIAN_POINT('',(129.8,-8.34768646165761,-31.9267306615923));
#25680=CARTESIAN_POINT('Origin',(129.6,0.,-6.66133814775094E-15));
#25681=CARTESIAN_POINT('',(129.8,-3.55817751859848,-14.0520399427901));
#25682=CARTESIAN_POINT('Origin',(125.8,-8.54102848838319,-31.8755522675393));
#25683=CARTESIAN_POINT('',(126.,-5.95283803735798,-22.2162940046486));
#25684=CARTESIAN_POINT('',(125.8,-5.95283803735798,-22.2162940046486));
#25685=CARTESIAN_POINT('',(126.,-8.54102848838319,-31.8755522675393));
#25686=CARTESIAN_POINT('',(126.,-2.83028733487431,-10.5627761337696));
#25687=CARTESIAN_POINT('',(125.8,-8.54102848838319,-31.8755522675393));
#25688=CARTESIAN_POINT('Origin',(125.9,-2.7336947522454,-10.5886580382799));
#25689=CARTESIAN_POINT('',(125.8,-8.34768646165762,-31.9267306615923));
#25690=CARTESIAN_POINT('Origin',(126.,0.,-6.66133814775094E-15));
#25691=CARTESIAN_POINT('',(125.8,-5.75942780780634,-22.2672178622896));
#25692=CARTESIAN_POINT('Origin',(126.,0.,0.));
#25693=CARTESIAN_POINT('',(125.8,-2.6371021696165,-10.6145399427901));
#25694=CARTESIAN_POINT('Origin',(129.7,-2.36067487571478,9.19652890683454));
#25695=CARTESIAN_POINT('',(129.8,-8.3476864616576,31.9267306615923));
#25696=CARTESIAN_POINT('',(129.6,-8.54102848838318,31.8755522675393));
#25697=CARTESIAN_POINT('Origin',(129.6,0.,-6.66133814775094E-15));
#25698=CARTESIAN_POINT('',(129.6,-5.95283803735798,22.2162940046486));
#25699=CARTESIAN_POINT('',(129.6,-2.45726745834369,9.17064700232429));
#25700=CARTESIAN_POINT('',(129.8,-5.75942780780634,22.2672178622896));
#25701=CARTESIAN_POINT('Origin',(129.6,0.,0.));
#25702=CARTESIAN_POINT('',(129.8,-2.26408229308588,9.22241081134479));
#25703=CARTESIAN_POINT('Origin',(125.8,-5.95283803735798,22.2162940046486));
#25704=CARTESIAN_POINT('',(126.,-8.54102848838318,31.8755522675393));
#25705=CARTESIAN_POINT('',(125.8,-8.54102848838318,31.8755522675393));
#25706=CARTESIAN_POINT('',(126.,-5.95283803735798,22.2162940046486));
#25707=CARTESIAN_POINT('',(126.,-1.53619210936171,5.73314700232429));
#25708=CARTESIAN_POINT('',(125.8,-5.95283803735798,22.2162940046486));
#25709=CARTESIAN_POINT('Origin',(125.9,-1.4395995267328,5.75902890683454));
#25710=CARTESIAN_POINT('',(125.8,-5.75942780780634,22.2672178622896));
#25711=CARTESIAN_POINT('Origin',(126.,0.,0.));
#25712=CARTESIAN_POINT('',(125.8,-8.34768646165761,31.9267306615923));
#25713=CARTESIAN_POINT('Origin',(126.,0.,-6.66133814775094E-15));
#25714=CARTESIAN_POINT('',(125.8,-1.3430069441039,5.78491081134479));
#25715=CARTESIAN_POINT('Origin',(125.8,0.,-6.66133814775094E-15));
#25716=CARTESIAN_POINT('Origin',(125.8,0.,-6.66133814775094E-15));
#25717=CARTESIAN_POINT('Origin',(129.8,0.,-6.66133814775094E-15));
#25718=CARTESIAN_POINT('Origin',(125.8,0.,0.));
#25719=CARTESIAN_POINT('Origin',(125.8,0.,0.));
#25720=CARTESIAN_POINT('Origin',(129.8,0.,0.));
#25721=CARTESIAN_POINT('Origin',(125.8,0.,4.44089209850063E-15));
#25722=CARTESIAN_POINT('Origin',(125.8,0.,4.44089209850063E-15));
#25723=CARTESIAN_POINT('Origin',(129.8,0.,4.44089209850063E-15));
#25724=CARTESIAN_POINT('Origin',(125.8,-2.22044604925031E-15,0.));
#25725=CARTESIAN_POINT('Origin',(125.8,-2.22044604925031E-15,0.));
#25726=CARTESIAN_POINT('Origin',(129.8,-2.22044604925031E-15,0.));
#25727=CARTESIAN_POINT('Origin',(127.8,0.,0.));
#25728=CARTESIAN_POINT('',(129.8,-15.5,-1.8982025386784E-15));
#25729=CARTESIAN_POINT('Origin',(129.8,0.,0.));
#25730=CARTESIAN_POINT('',(125.8,-15.5,-1.8982025386784E-15));
#25731=CARTESIAN_POINT('',(127.8,-15.5,-1.8982025386784E-15));
#25732=CARTESIAN_POINT('Origin',(125.8,0.,0.));
#25733=CARTESIAN_POINT('Origin',(125.8,43.,0.));
#25734=CARTESIAN_POINT('',(125.8,-43.,-5.26598123633362E-15));
#25735=CARTESIAN_POINT('Origin',(125.8,0.,0.));
#25736=CARTESIAN_POINT('Origin',(127.8,0.,0.));
#25737=CARTESIAN_POINT('',(129.8,-43.,-5.26598123633362E-15));
#25738=CARTESIAN_POINT('Origin',(129.8,0.,0.));
#25739=CARTESIAN_POINT('',(127.8,-43.,-5.26598123633362E-15));
#25740=CARTESIAN_POINT('Origin',(129.8,15.5,0.));
#38479=UNCERTAINTY_MEASURE_WITH_UNIT(LENGTH_MEASURE(0.01),#38508,
'DISTANCE_ACCURACY_VALUE',
'Maximum model space distance between geometric entities at asserted c
onnectivities');
#38490=UNCERTAINTY_MEASURE_WITH_UNIT(LENGTH_MEASURE(0.01),#38508,
'DISTANCE_ACCURACY_VALUE',
'Maximum model space distance between geometric entities at asserted c
onnectivities');
#38496=(
GEOMETRIC_REPRESENTATION_CONTEXT(3)
GLOBAL_UNCERTAINTY_ASSIGNED_CONTEXT((#38479))
GLOBAL_UNIT_ASSIGNED_CONTEXT((#38508,#38510,#38511))
REPRESENTATION_CONTEXT('','3D')
);
#38507=(
GEOMETRIC_REPRESENTATION_CONTEXT(3)
GLOBAL_UNCERTAINTY_ASSIGNED_CONTEXT((#38490))
GLOBAL_UNIT_ASSIGNED_CONTEXT((#38508,#38510,#38511))
REPRESENTATION_CONTEXT('','3D')
);
#38508=(
LENGTH_UNIT()
NAMED_UNIT(*)
SI_UNIT(.MILLI.,.METRE.)
);
#38510=(
NAMED_UNIT(*)
PLANE_ANGLE_UNIT()
SI_UNIT($,.RADIAN.)
);
#38511=(
NAMED_UNIT(*)
SI_UNIT($,.STERADIAN.)
SOLID_ANGLE_UNIT()
);
#38517=SHAPE_DEFINITION_REPRESENTATION(#38533,#38579);
#38533=PRODUCT_DEFINITION_SHAPE('',$,#38596);
#38579=SHAPE_REPRESENTATION('',(#15901),#38496);
#38590=PRODUCT_DEFINITION_CONTEXT('part definition',#38640,'design');
#38596=PRODUCT_DEFINITION('2026-10-26-01-10-50-811','08_Valve_Plate',#38612,
#38590);
#38612=PRODUCT_DEFINITION_FORMATION('',$,#38647);
#38640=APPLICATION_CONTEXT(
'Core Data for Automotive Mechanical Design Process');
#38641=PRODUCT_CONTEXT('part definition',#38640,'mechanical');
#38647=PRODUCT('2026-10-26-01-10-50-811','08_Valve_Plate',$,(#38641));
#38700=COLOUR_RGB('Light Blue',0.38,0.62,0.78);
#38701=FILL_AREA_STYLE_COLOUR('',#38700);
#38702=FILL_AREA_STYLE('',(#38701));
#38703=SURFACE_STYLE_FILL_AREA(#38702);
#38704=SURFACE_SIDE_STYLE('',(#38703));
#38705=SURFACE_STYLE_USAGE(.BOTH.,#38704);
#38706=PRESENTATION_STYLE_ASSIGNMENT((#38705));
ENDSEC;
END-ISO-10303-21;
